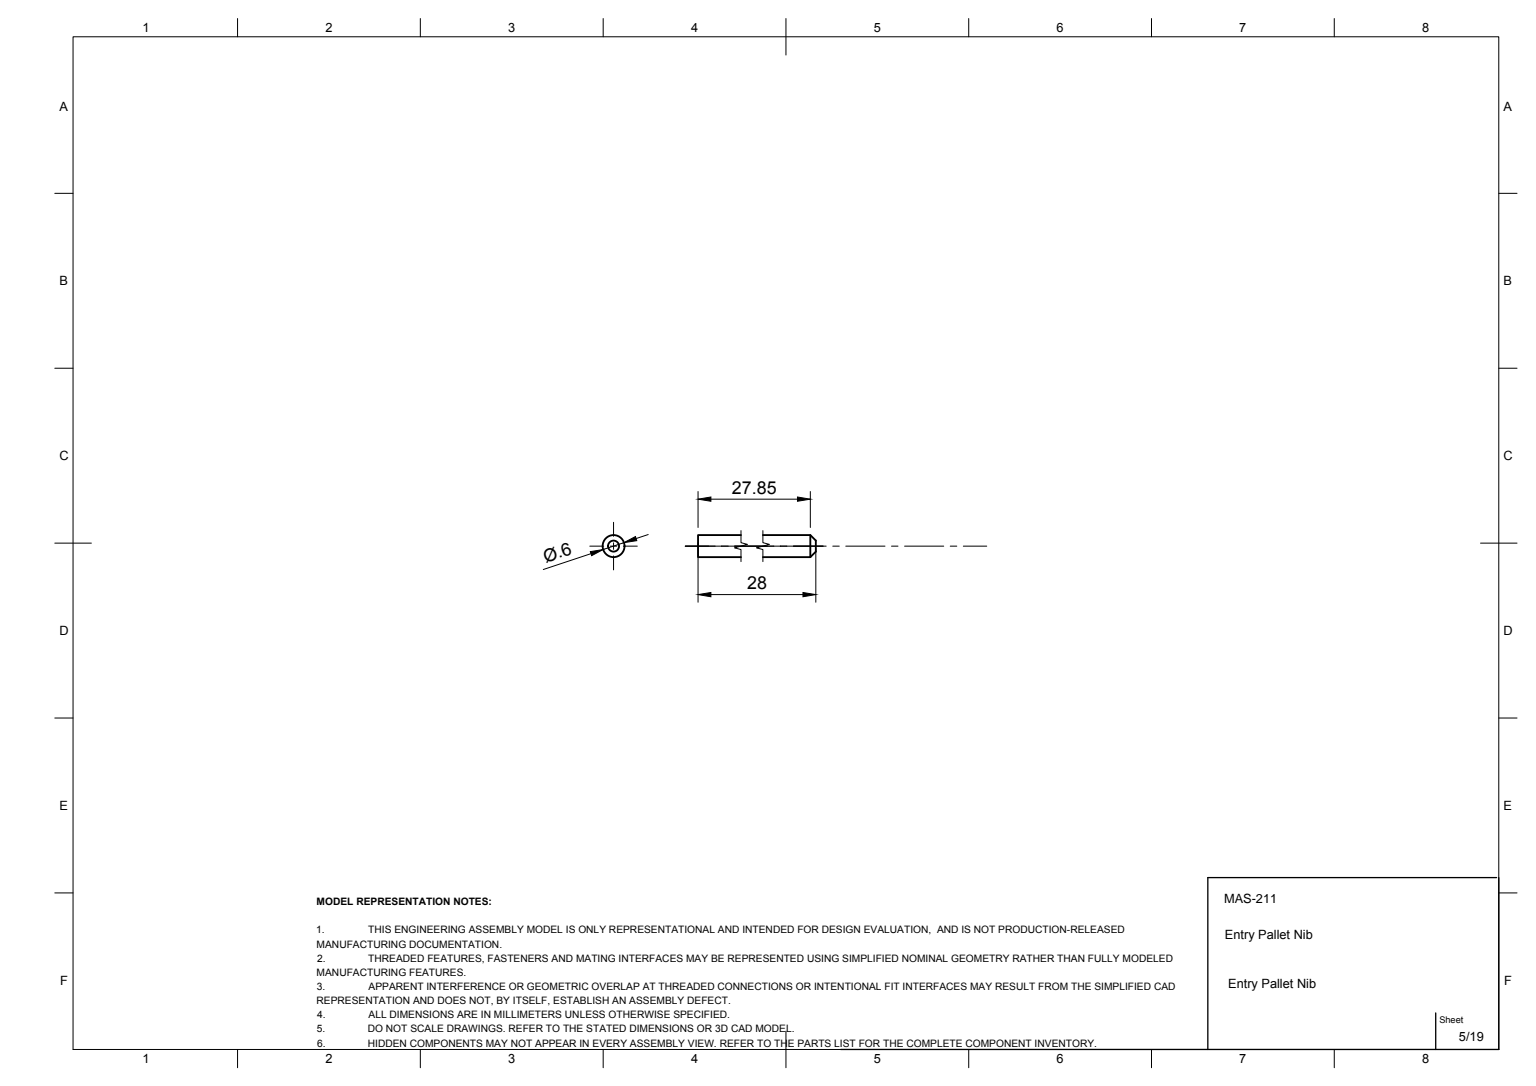
ISO-10303-21;
HEADER;
FILE_DESCRIPTION(
 (''),
 '2;1');
FILE_NAME ( 'Entry Pallet Nib.step', '2026-10-05T20:07:59+06:00', ( '' ), ( '' ), 'STEP AP214', 'Unspecified', '' );
FILE_SCHEMA (('AUTOMOTIVE_DESIGN { 1 0 10303 214 3 1 1 }'));
ENDSEC;
DATA;
#10=MECHANICAL_DESIGN_GEOMETRIC_PRESENTATION_REPRESENTATION('',(#321),#196741);
#321=STYLED_ITEM('',(#196765),#340) ;
#340=MANIFOLD_SOLID_BREP('Entry Pallet Nib',#8717) ;
#365=PLANE('',#8798) ;
#366=PLANE('',#8799) ;
#626=CIRCLE('',#8795,0.299999999999999) ;
#627=CIRCLE('',#8796,0.300000000000007) ;
#628=CIRCLE('',#8797,0.300000000000007) ;
#831=B_SPLINE_SURFACE_WITH_KNOTS('',3,1,((#79282,#79283),(#79284,#79285),
(#79286,#79287),(#79288,#79289),(#79290,#79291),(#79292,#79293),(#79294,
#79295),(#79296,#79297),(#79298,#79299),(#79300,#79301),(#79302,#79303)),
 .UNSPECIFIED.,.T.,.F.,.F.,(4,1,1,1,1,1,1,1,4),(2,2),(0.,0.117806748710524,
0.235613497421048,0.353420242239986,0.471226987058923,0.58903373187812,
0.706840476697317,0.824647225407855,0.942453974118393),(0.,0.239984718977347),
 .UNSPECIFIED.) ;
#911=FACE_OUTER_BOUND('',#1394,.T.) ;
#912=FACE_OUTER_BOUND('',#1395,.T.) ;
#913=FACE_OUTER_BOUND('',#1396,.T.) ;
#914=FACE_OUTER_BOUND('',#1397,.T.) ;
#1394=EDGE_LOOP('',(#5884,#5885,#5886,#5887,#5888)) ;
#1395=EDGE_LOOP('',(#5889)) ;
#1396=EDGE_LOOP('',(#5890)) ;
#1397=EDGE_LOOP('',(#5891,#5892,#5893,#5894,#5895)) ;
#1903=LINE('',#79264,#2606) ;
#1904=LINE('',#79304,#2607) ;
#2606=VECTOR('',#9595,0.299999999999991) ;
#2607=VECTOR('',#9604,10.) ;
#3373=B_SPLINE_CURVE_WITH_KNOTS('',3,(#79271,#79272,#79273,#79274,#79275,
#79276,#79277,#79278,#79279,#79280,#79281),.UNSPECIFIED.,.T.,.F.,(4,1,1,
1,1,1,1,1,4),(0.,0.117806748710524,0.235613497421048,0.353420242239986,
0.471226987058923,0.58903373187812,0.706840476697317,0.824647225407855,
0.942453974118393),.UNSPECIFIED.) ;
#3555=VERTEX_POINT('',#79261) ;
#3556=VERTEX_POINT('',#79263) ;
#3557=VERTEX_POINT('',#79265) ;
#3558=VERTEX_POINT('',#79270) ;
#4450=EDGE_CURVE('',#3555,#3555,#626,.T.) ;
#4451=EDGE_CURVE('',#3555,#3556,#1903,.T.) ;
#4452=EDGE_CURVE('',#3557,#3556,#627,.T.) ;
#4453=EDGE_CURVE('',#3556,#3557,#628,.T.) ;
#4454=EDGE_CURVE('',#3558,#3558,#3373,.T.) ;
#4455=EDGE_CURVE('',#3557,#3558,#1904,.T.) ;
#5884=ORIENTED_EDGE('',*,*,#4450,.F.) ;
#5885=ORIENTED_EDGE('',*,*,#4451,.T.) ;
#5886=ORIENTED_EDGE('',*,*,#4452,.F.) ;
#5887=ORIENTED_EDGE('',*,*,#4453,.F.) ;
#5888=ORIENTED_EDGE('',*,*,#4451,.F.) ;
#5889=ORIENTED_EDGE('',*,*,#4450,.T.) ;
#5890=ORIENTED_EDGE('',*,*,#4454,.T.) ;
#5891=ORIENTED_EDGE('',*,*,#4452,.T.) ;
#5892=ORIENTED_EDGE('',*,*,#4453,.T.) ;
#5893=ORIENTED_EDGE('',*,*,#4455,.T.) ;
#5894=ORIENTED_EDGE('',*,*,#4454,.F.) ;
#5895=ORIENTED_EDGE('',*,*,#4455,.F.) ;
#8142=CYLINDRICAL_SURFACE('',#8794,0.299999999999991) ;
#8294=ADVANCED_FACE('',(#911),#8142,.T.) ;
#8295=ADVANCED_FACE('',(#912),#365,.T.) ;
#8296=ADVANCED_FACE('',(#913),#366,.T.) ;
#8297=ADVANCED_FACE('',(#914),#831,.T.) ;
#8717=CLOSED_SHELL('',(#8294,#8295,#8296,#8297)) ;
#8794=AXIS2_PLACEMENT_3D('',#79260,#9591,#9592) ;
#8795=AXIS2_PLACEMENT_3D('',#79262,#9593,#9594) ;
#8796=AXIS2_PLACEMENT_3D('',#79266,#9596,#9597) ;
#8797=AXIS2_PLACEMENT_3D('',#79267,#9598,#9599) ;
#8798=AXIS2_PLACEMENT_3D('',#79268,#9600,#9601) ;
#8799=AXIS2_PLACEMENT_3D('',#79269,#9602,#9603) ;
#9591=DIRECTION('center_axis',(0.946101641249535,-1.74964368949631E-30,
0.323869857234254)) ;
#9592=DIRECTION('ref_axis',(-1.69501880657431E-15,1.,0.)) ;
#9593=DIRECTION('center_axis',(0.946101641249537,1.59018832135268E-14,0.323869857234249)) ;
#9594=DIRECTION('ref_axis',(0.188203553203261,0.813826036051114,-0.549787782336964)) ;
#9595=DIRECTION('',(-0.946101641249535,1.74964368949631E-30,-0.323869857234254)) ;
#9596=DIRECTION('center_axis',(-0.946101641249539,-4.86663357488556E-15,
-0.323869857234242)) ;
#9597=DIRECTION('ref_axis',(-0.188203553203284,0.813826036051079,0.54978778233701)) ;
#9598=DIRECTION('center_axis',(-0.946101641249539,-4.86663357488556E-15,
-0.323869857234242)) ;
#9599=DIRECTION('ref_axis',(-0.188203553203284,0.813826036051079,0.54978778233701)) ;
#9600=DIRECTION('center_axis',(0.946101641249535,0.,0.323869857234254)) ;
#9601=DIRECTION('ref_axis',(0.323869857234254,0.,-0.946101641249535)) ;
#9602=DIRECTION('center_axis',(-0.946101641249535,-1.97215226305253E-31,
-0.323869857234254)) ;
#9603=DIRECTION('ref_axis',(-0.323869857234254,0.,0.946101641249535)) ;
#9604=DIRECTION('',(-0.668994894197647,-0.707106772753729,-0.229010575003176)) ;
#79260=CARTESIAN_POINT('Origin',(-5.63784594070025E-6,12.,130.056019952763)) ;
#79261=CARTESIAN_POINT('',(3.7844009271522,11.7,131.3514993817)) ;
#79262=CARTESIAN_POINT('Origin',(3.7844009271522,12.,131.3514993817)) ;
#79263=CARTESIAN_POINT('',(-22.5645297816473,11.7,122.331723857726)) ;
#79264=CARTESIAN_POINT('',(-5.63784594017984E-6,11.7,130.056019952763)) ;
#79265=CARTESIAN_POINT('',(-22.5645297816474,12.3,122.331723857726)) ;
#79266=CARTESIAN_POINT('Origin',(-22.5645297816474,12.,122.331723857726)) ;
#79267=CARTESIAN_POINT('Origin',(-22.5645297816474,12.,122.331723857726)) ;
#79268=CARTESIAN_POINT('Origin',(6.05149556563793,0.999999999999999,124.728771423451)) ;
#79269=CARTESIAN_POINT('Origin',(-22.7064450278348,12.3,122.283143379141)) ;
#79270=CARTESIAN_POINT('',(-22.7064450278348,12.1500000035778,122.283143379141)) ;
#79271=CARTESIAN_POINT('Ctrl Pts',(-22.7064450278348,12.1500000035778,122.283143379141)) ;
#79272=CARTESIAN_POINT('Ctrl Pts',(-22.6937453390508,12.1502314747086,122.246044537944)) ;
#79273=CARTESIAN_POINT('Ctrl Pts',(-22.6683574552983,12.1175431645324,122.171880431747)) ;
#79274=CARTESIAN_POINT('Ctrl Pts',(-22.6525723366187,12.0000444315862,122.125768308755)) ;
#79275=CARTESIAN_POINT('Ctrl Pts',(-22.6683514162181,11.8823598076173,122.171862790143)) ;
#79276=CARTESIAN_POINT('Ctrl Pts',(-22.7064423304138,11.8336812214274,122.283135499326)) ;
#79277=CARTESIAN_POINT('Ctrl Pts',(-22.7445380204197,11.8823694052799,122.394422159798)) ;
#79278=CARTESIAN_POINT('Ctrl Pts',(-22.7603151873203,12.0000313447684,122.440511053734)) ;
#79279=CARTESIAN_POINT('Ctrl Pts',(-22.74452995505,12.1175454374094,122.394398598916)) ;
#79280=CARTESIAN_POINT('Ctrl Pts',(-22.7191521346486,12.1502048378774,122.320263890184)) ;
#79281=CARTESIAN_POINT('Ctrl Pts',(-22.7064450278348,12.1500000035778,122.283143379141)) ;
#79282=CARTESIAN_POINT('Ctrl Pts',(-22.5645297816474,12.3,122.331723857726)) ;
#79283=CARTESIAN_POINT('Ctrl Pts',(-22.7064450278348,12.1500000035778,122.283143379141)) ;
#79284=CARTESIAN_POINT('Ctrl Pts',(-22.5391304026157,12.3004629406991,122.257526171057)) ;
#79285=CARTESIAN_POINT('Ctrl Pts',(-22.6937453390508,12.1502314747086,122.246044537944)) ;
#79286=CARTESIAN_POINT('Ctrl Pts',(-22.4883546371039,12.2350863374522,122.109197964485)) ;
#79287=CARTESIAN_POINT('Ctrl Pts',(-22.6683574552983,12.1175431645324,122.171880431747)) ;
#79288=CARTESIAN_POINT('Ctrl Pts',(-22.456784402798,12.0000888605178,122.016973727421)) ;
#79289=CARTESIAN_POINT('Ctrl Pts',(-22.6525723366187,12.0000444315862,122.125768308755)) ;
#79290=CARTESIAN_POINT('Ctrl Pts',(-22.4883425568402,11.7647196121379,122.109162675133)) ;
#79291=CARTESIAN_POINT('Ctrl Pts',(-22.6683514162181,11.8823598076173,122.171862790143)) ;
#79292=CARTESIAN_POINT('Ctrl Pts',(-22.5645243863183,11.6673624555447,122.331708096674)) ;
#79293=CARTESIAN_POINT('Ctrl Pts',(-22.7064423304138,11.8336812214274,122.283135499326)) ;
#79294=CARTESIAN_POINT('Ctrl Pts',(-22.6407157694817,11.7647388086052,122.554281426824)) ;
#79295=CARTESIAN_POINT('Ctrl Pts',(-22.7445380204197,11.8823694052799,122.394422159798)) ;
#79296=CARTESIAN_POINT('Ctrl Pts',(-22.6722700958943,12.0000626848499,122.646459193111)) ;
#79297=CARTESIAN_POINT('Ctrl Pts',(-22.7603151873203,12.0000313447684,122.440511053734)) ;
#79298=CARTESIAN_POINT('Ctrl Pts',(-22.640699636509,12.2350908868498,122.554234298536)) ;
#79299=CARTESIAN_POINT('Ctrl Pts',(-22.74452995505,12.1175454374094,122.394398598916)) ;
#79300=CARTESIAN_POINT('Ctrl Pts',(-22.5899439964264,12.3004096643473,122.405964883176)) ;
#79301=CARTESIAN_POINT('Ctrl Pts',(-22.7191521346486,12.1502048378774,122.320263890184)) ;
#79302=CARTESIAN_POINT('Ctrl Pts',(-22.5645297816474,12.3,122.331723857726)) ;
#79303=CARTESIAN_POINT('Ctrl Pts',(-22.7064450278348,12.1500000035778,122.283143379141)) ;
#79304=CARTESIAN_POINT('',(-22.5645297816474,12.3,122.331723857726)) ;
#196737=UNCERTAINTY_MEASURE_WITH_UNIT(LENGTH_MEASURE(0.01),#196742,
'DISTANCE_ACCURACY_VALUE',
'Maximum model space distance between geometric entities at asserted c
onnectivities') ;
#196738=UNCERTAINTY_MEASURE_WITH_UNIT(LENGTH_MEASURE(0.01),#196742,
'DISTANCE_ACCURACY_VALUE',
'Maximum model space distance between geometric entities at asserted c
onnectivities') ;
#196740=(
GEOMETRIC_REPRESENTATION_CONTEXT(3)
GLOBAL_UNCERTAINTY_ASSIGNED_CONTEXT((#196737))
GLOBAL_UNIT_ASSIGNED_CONTEXT((#196742,#196744,#196745))
REPRESENTATION_CONTEXT('','3D')
) ;
#196741=(
GEOMETRIC_REPRESENTATION_CONTEXT(3)
GLOBAL_UNCERTAINTY_ASSIGNED_CONTEXT((#196738))
GLOBAL_UNIT_ASSIGNED_CONTEXT((#196742,#196744,#196745))
REPRESENTATION_CONTEXT('','3D')
) ;
#196742=(
LENGTH_UNIT()
NAMED_UNIT(*)
SI_UNIT(.MILLI.,.METRE.)
) ;
#196744=(
NAMED_UNIT(*)
PLANE_ANGLE_UNIT()
SI_UNIT($,.RADIAN.)
) ;
#196745=(
NAMED_UNIT(*)
SI_UNIT($,.STERADIAN.)
SOLID_ANGLE_UNIT()
) ;
#196753=PRODUCT_DEFINITION_CONTEXT('part definition',#196761,'design') ;
#196761=APPLICATION_CONTEXT(
'Core Data for Automotive Mechanical Design Process') ;
#196762=PRODUCT_CONTEXT('part definition',#196761,'mechanical') ;
#196765=PRESENTATION_STYLE_ASSIGNMENT((#196767)) ;
#196767=SURFACE_STYLE_USAGE(.BOTH.,#196769) ;
#196769=SURFACE_SIDE_STYLE('',(#196771)) ;
#196771=SURFACE_STYLE_FILL_AREA(#196773) ;
#196773=FILL_AREA_STYLE('Steel - Satin',(#196775)) ;
#196775=FILL_AREA_STYLE_COLOUR('Steel - Satin',#196777) ;
#196777=COLOUR_RGB('Steel - Satin', 0.09019608, 0.27058824, 0.51372549) ;
#196827=CARTESIAN_POINT ( '', ( 0.0, 0.0, 0.0 ) ) ;
#196828=DIRECTION ( '', ( 0.0, 0.0, 1.0 ) ) ;
#196829=DIRECTION ( '', ( 1.0, 0.0, 0.0 ) ) ;
#196830=AXIS2_PLACEMENT_3D ( '', #196827, #196828, #196829 ) ;
#196831=ADVANCED_BREP_SHAPE_REPRESENTATION ( 'Entry Pallet Nib', ( #340, #196830, #196841, #197264 ), #196740 ) ;
#196832=PRODUCT( 'Entry Pallet Nib', 'Entry Pallet Nib', '', ( #196762 ) ) ;
#196833=PRODUCT_DEFINITION_FORMATION ( '', '', #196832 ) ;
#196834=PRODUCT_DEFINITION( 'Entry Pallet Nib', 'Entry Pallet Nib', #196833, #196753 ) ;
#196835=PRODUCT_DEFINITION_SHAPE ( '', '', #196834 ) ;
#196836=SHAPE_DEFINITION_REPRESENTATION ( #196835, #196831 ) ;
#196838=CARTESIAN_POINT ( '', ( 0.0, 0.0, 0.0 ) ) ;
#196839=DIRECTION ( '', ( 0.0, 0.0, 1.0 ) ) ;
#196840=DIRECTION ( '', ( 1.0, 0.0, 0.0 ) ) ;
#196841=AXIS2_PLACEMENT_3D ( '', #196838, #196839, #196840 ) ;
#197261=CARTESIAN_POINT ( '', ( 0.0, 0.0, 0.0 ) ) ;
#197262=DIRECTION ( '', ( 0.0, 0.0, 1.0 ) ) ;
#197263=DIRECTION ( '', ( 1.0, 0.0, 0.0 ) ) ;
#197264=AXIS2_PLACEMENT_3D ( '', #197261, #197262, #197263 ) ;
ENDSEC;
END-ISO-10303-21;
